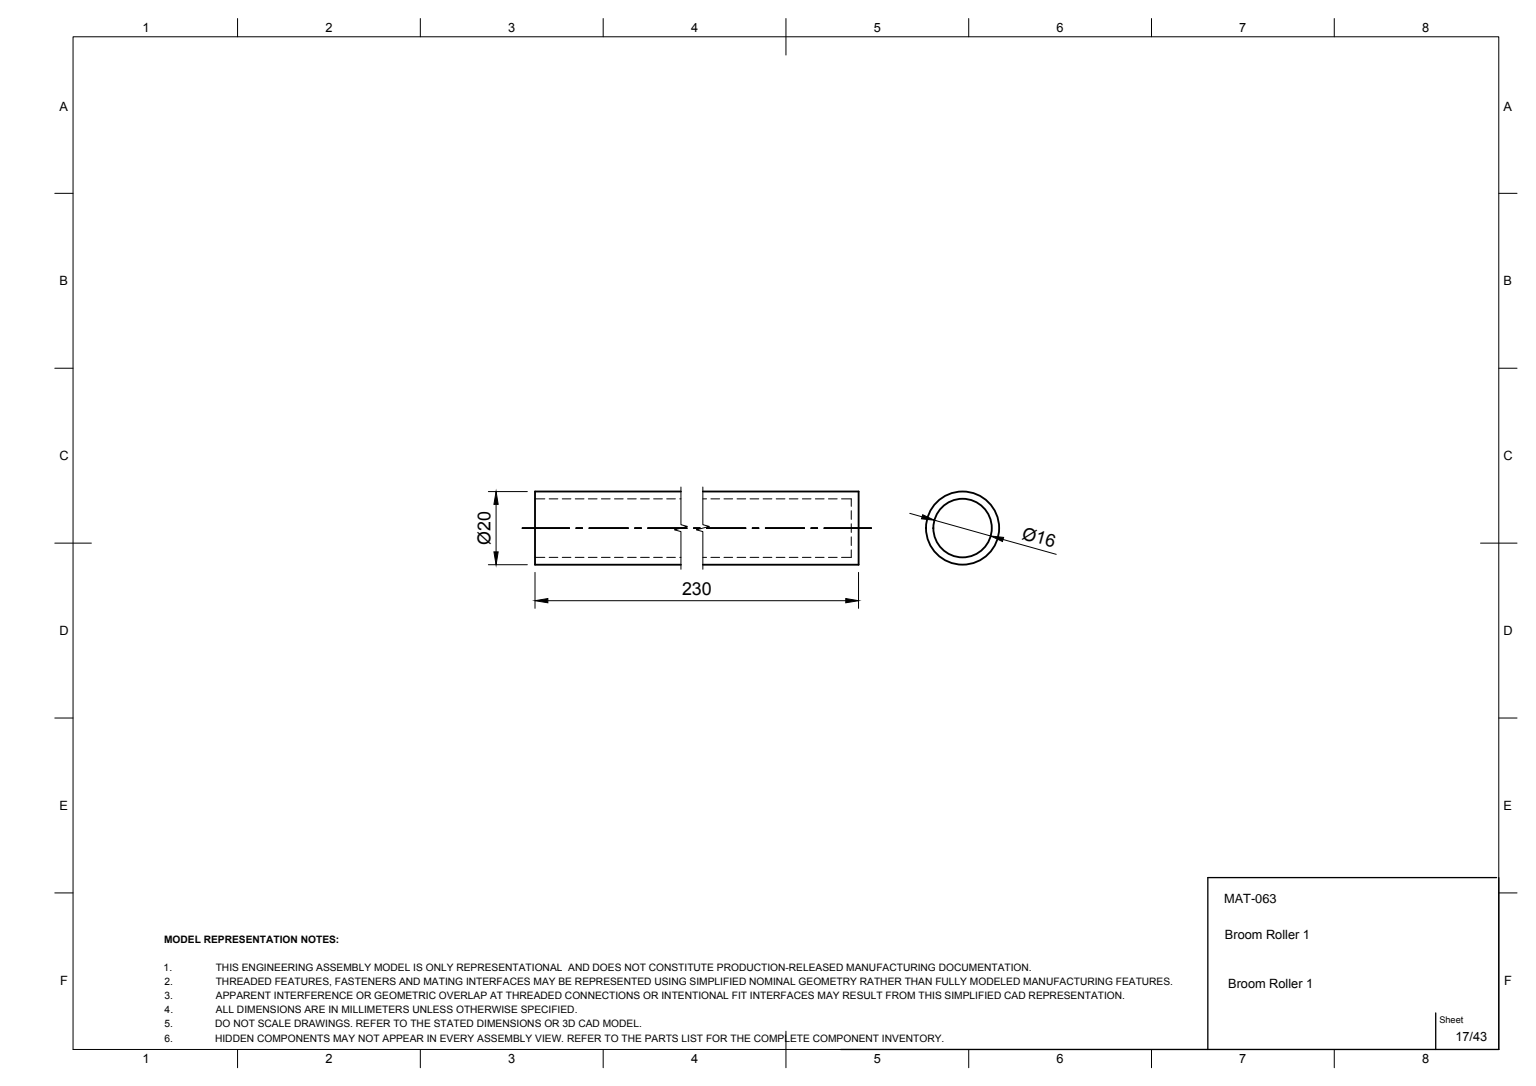
ISO-10303-21;
HEADER;
/* Generated by software containing ST-Developer
 * from STEP Tools, Inc. (www.steptools.com) 
 */

FILE_DESCRIPTION(
/* description */ (''),
/* implementation_level */ '2;1');

FILE_NAME(
/* name */ 'Broom Roller 1.step',
/* time_stamp */ '2026-10-24T09:43:01-07:00',
/* author */ (''),
/* organization */ (''),
/* preprocessor_version */ 'ST-DEVELOPER v20.2',
/* originating_system */ 'Autodesk Translation Framework v15.15.0.0',
/* authorisation */ '');

FILE_SCHEMA (('AUTOMOTIVE_DESIGN { 1 0 10303 214 3 1 1 }'));
ENDSEC;

DATA;
#10=MECHANICAL_DESIGN_GEOMETRIC_PRESENTATION_REPRESENTATION('',(#282),#11112);
#216=SHAPE_REPRESENTATION_RELATIONSHIP('SRR','None',#11240,#249);
#249=ADVANCED_BREP_SHAPE_REPRESENTATION('',(#315),#11085);
#282=STYLED_ITEM('',(#11426),#315);
#315=MANIFOLD_SOLID_BREP('Broom Roller 1',#6019);
#412=FACE_BOUND('',#1277,.T.);
#543=PLANE('',#6832);
#544=PLANE('',#6833);
#545=PLANE('',#6837);
#837=FACE_OUTER_BOUND('',#1274,.T.);
#838=FACE_OUTER_BOUND('',#1275,.T.);
#839=FACE_OUTER_BOUND('',#1276,.T.);
#840=FACE_OUTER_BOUND('',#1278,.T.);
#841=FACE_OUTER_BOUND('',#1279,.T.);
#1274=EDGE_LOOP('',(#4667,#4668,#4669,#4670));
#1275=EDGE_LOOP('',(#4671));
#1276=EDGE_LOOP('',(#4672));
#1277=EDGE_LOOP('',(#4673));
#1278=EDGE_LOOP('',(#4674,#4675,#4676,#4677));
#1279=EDGE_LOOP('',(#4678));
#1669=LINE('',#10088,#2028);
#1670=LINE('',#10097,#2029);
#2028=VECTOR('',#8219,0.00799999973819874);
#2029=VECTOR('',#8232,0.00999999988959839);
#2522=CIRCLE('',#6830,0.00799999973819874);
#2523=CIRCLE('',#6831,0.00799999973819874);
#2524=CIRCLE('',#6834,0.00999999988959839);
#2525=CIRCLE('',#6836,0.00999999988959839);
#2908=VERTEX_POINT('',#10085);
#2909=VERTEX_POINT('',#10087);
#2910=VERTEX_POINT('',#10092);
#2911=VERTEX_POINT('',#10095);
#3537=EDGE_CURVE('',#2908,#2908,#2522,.T.);
#3538=EDGE_CURVE('',#2908,#2909,#1669,.T.);
#3539=EDGE_CURVE('',#2909,#2909,#2523,.F.);
#3540=EDGE_CURVE('',#2910,#2910,#2524,.T.);
#3541=EDGE_CURVE('',#2911,#2911,#2525,.F.);
#3542=EDGE_CURVE('',#2911,#2910,#1670,.T.);
#4667=ORIENTED_EDGE('',*,*,#3537,.F.);
#4668=ORIENTED_EDGE('',*,*,#3538,.T.);
#4669=ORIENTED_EDGE('',*,*,#3539,.F.);
#4670=ORIENTED_EDGE('',*,*,#3538,.F.);
#4671=ORIENTED_EDGE('',*,*,#3539,.T.);
#4672=ORIENTED_EDGE('',*,*,#3540,.F.);
#4673=ORIENTED_EDGE('',*,*,#3537,.T.);
#4674=ORIENTED_EDGE('',*,*,#3541,.T.);
#4675=ORIENTED_EDGE('',*,*,#3542,.T.);
#4676=ORIENTED_EDGE('',*,*,#3540,.T.);
#4677=ORIENTED_EDGE('',*,*,#3542,.F.);
#4678=ORIENTED_EDGE('',*,*,#3541,.F.);
#5568=CYLINDRICAL_SURFACE('',#6829,0.00799999973819874);
#5569=CYLINDRICAL_SURFACE('',#6835,0.00999999988959839);
#5810=ADVANCED_FACE('',(#837),#5568,.F.);
#5811=ADVANCED_FACE('',(#838),#543,.F.);
#5812=ADVANCED_FACE('',(#839,#412),#544,.F.);
#5813=ADVANCED_FACE('',(#840),#5569,.T.);
#5814=ADVANCED_FACE('',(#841),#545,.T.);
#6019=CLOSED_SHELL('',(#5810,#5811,#5812,#5813,#5814));
#6828=AXIS2_PLACEMENT_3D('',#10083,#8213,#8214);
#6829=AXIS2_PLACEMENT_3D('',#10084,#8215,#8216);
#6830=AXIS2_PLACEMENT_3D('',#10086,#8217,#8218);
#6831=AXIS2_PLACEMENT_3D('',#10089,#8220,#8221);
#6832=AXIS2_PLACEMENT_3D('',#10090,#8222,#8223);
#6833=AXIS2_PLACEMENT_3D('',#10091,#8224,#8225);
#6834=AXIS2_PLACEMENT_3D('',#10093,#8226,#8227);
#6835=AXIS2_PLACEMENT_3D('',#10094,#8228,#8229);
#6836=AXIS2_PLACEMENT_3D('',#10096,#8230,#8231);
#6837=AXIS2_PLACEMENT_3D('',#10098,#8233,#8234);
#8213=DIRECTION('axis',(0.,0.,1.));
#8214=DIRECTION('refdir',(1.,0.,0.));
#8215=DIRECTION('center_axis',(0.,0.992193411636613,-0.124708595954326));
#8216=DIRECTION('ref_axis',(0.,0.124708595954326,0.992193411636613));
#8217=DIRECTION('center_axis',(0.,0.992193411636613,-0.124708595954326));
#8218=DIRECTION('ref_axis',(0.,0.124708595954326,0.992193411636613));
#8219=DIRECTION('',(0.,0.992193411636613,-0.124708595954326));
#8220=DIRECTION('center_axis',(0.,0.992193411636613,-0.124708595954326));
#8221=DIRECTION('ref_axis',(0.,0.124708595954326,0.992193411636613));
#8222=DIRECTION('center_axis',(1.04435470755135E-16,0.992193408738347,-0.124708619013202));
#8223=DIRECTION('ref_axis',(9.66752478783401E-35,0.124708619013202,0.992193408738347));
#8224=DIRECTION('center_axis',(2.63594069435475E-16,0.992193411026652,-0.124708600807231));
#8225=DIRECTION('ref_axis',(-6.9705924208555E-34,0.124708600807231,0.992193411026652));
#8226=DIRECTION('center_axis',(0.,0.992193411636614,-0.124708595954319));
#8227=DIRECTION('ref_axis',(0.,0.124708595954319,0.992193411636613));
#8228=DIRECTION('center_axis',(0.,0.992193411636614,-0.124708595954319));
#8229=DIRECTION('ref_axis',(0.,0.124708595954319,0.992193411636613));
#8230=DIRECTION('center_axis',(0.,0.992193411636614,-0.124708595954319));
#8231=DIRECTION('ref_axis',(0.,0.124708595954319,0.992193411636613));
#8232=DIRECTION('',(0.,-0.992193411636613,0.124708595954319));
#8233=DIRECTION('center_axis',(2.38185692356041E-15,0.992193411026652,-0.124708600807233));
#8234=DIRECTION('ref_axis',(-6.67137153928239E-35,0.124708600807233,0.992193411026652));
#10083=CARTESIAN_POINT('',(0.,0.,0.));
#10084=CARTESIAN_POINT('Origin',(0.,0.121795515,1.128682977));
#10085=CARTESIAN_POINT('',(-9.79717407256475E-19,0.120797846530031,1.12074542993335));
#10086=CARTESIAN_POINT('Origin',(0.,0.121795515265017,1.12868297696669));
#10087=CARTESIAN_POINT('',(-9.79717407256475E-19,0.347017944542894,1.09231187003569));
#10088=CARTESIAN_POINT('',(-9.79717407256475E-19,0.120797846265014,1.12074542996666));
#10089=CARTESIAN_POINT('Origin',(0.,0.34801561327788,1.10024941706903));
#10090=CARTESIAN_POINT('Origin',(-1.99493199737333E-19,0.348015613,1.100249417));
#10091=CARTESIAN_POINT('Origin',(-1.56125112837913E-19,0.121795515,1.128682977));
#10092=CARTESIAN_POINT('',(-1.22464678562706E-18,0.120548429108451,1.11876104298636));
#10093=CARTESIAN_POINT('Origin',(0.,0.121795515054226,1.12868297699318));
#10094=CARTESIAN_POINT('Origin',(0.,0.121795515,1.128682977));
#10095=CARTESIAN_POINT('',(-1.22464678562706E-18,0.34875291409482,1.09007806587791));
#10096=CARTESIAN_POINT('Origin',(0.,0.350000000040595,1.09999999988473));
#10097=CARTESIAN_POINT('',(-1.22464678562706E-18,0.120548429054225,1.11876104299317));
#10098=CARTESIAN_POINT('Origin',(-1.56125112837913E-19,0.35,1.1));
#11046=UNCERTAINTY_MEASURE_WITH_UNIT(LENGTH_MEASURE(1.E-5),#11113,
'DISTANCE_ACCURACY_VALUE',
'Maximum model space distance between geometric entities at asserted c
onnectivities');
#11073=UNCERTAINTY_MEASURE_WITH_UNIT(LENGTH_MEASURE(1.E-5),#11113,
'DISTANCE_ACCURACY_VALUE',
'Maximum model space distance between geometric entities at asserted c
onnectivities');
#11085=(
GEOMETRIC_REPRESENTATION_CONTEXT(3)
GLOBAL_UNCERTAINTY_ASSIGNED_CONTEXT((#11046))
GLOBAL_UNIT_ASSIGNED_CONTEXT((#11113,#11114,#11115))
REPRESENTATION_CONTEXT('','3D')
);
#11112=(
GEOMETRIC_REPRESENTATION_CONTEXT(3)
GLOBAL_UNCERTAINTY_ASSIGNED_CONTEXT((#11073))
GLOBAL_UNIT_ASSIGNED_CONTEXT((#11113,#11114,#11115))
REPRESENTATION_CONTEXT('','3D')
);
#11113=(
LENGTH_UNIT()
NAMED_UNIT(*)
SI_UNIT($,.METRE.)
);
#11114=(
NAMED_UNIT(*)
PLANE_ANGLE_UNIT()
SI_UNIT($,.RADIAN.)
);
#11115=(
NAMED_UNIT(*)
SI_UNIT($,.STERADIAN.)
SOLID_ANGLE_UNIT()
);
#11127=SHAPE_DEFINITION_REPRESENTATION(#11165,#11240);
#11165=PRODUCT_DEFINITION_SHAPE('',$,#11279);
#11240=SHAPE_REPRESENTATION('',(#6828),#11085);
#11267=PRODUCT_DEFINITION_CONTEXT('part definition',#11383,'design');
#11279=PRODUCT_DEFINITION('Broom Roller 1','Broom Roller 1',#11317,#11267);
#11317=PRODUCT_DEFINITION_FORMATION('',$,#11396);
#11383=APPLICATION_CONTEXT(
'Core Data for Automotive Mechanical Design Process');
#11384=PRODUCT_CONTEXT('part definition',#11383,'mechanical');
#11396=PRODUCT('Broom Roller 1','Broom Roller 1',
'broom_and_roller__ DE     7425',(#11384));
#11426=PRESENTATION_STYLE_ASSIGNMENT((#11430));
#11430=SURFACE_STYLE_USAGE(.BOTH.,#11434);
#11434=SURFACE_SIDE_STYLE('',(#11438));
#11438=SURFACE_STYLE_FILL_AREA(#11442);
#11442=FILL_AREA_STYLE('Opaque(202,209,238)',(#11446));
#11446=FILL_AREA_STYLE_COLOUR('Opaque(202,209,238)',#11450);
#11450=COLOUR_RGB('Opaque(202,209,238)',0.792156862745098,0.819607843137255,
0.933333333333333);
ENDSEC;
END-ISO-10303-21;
